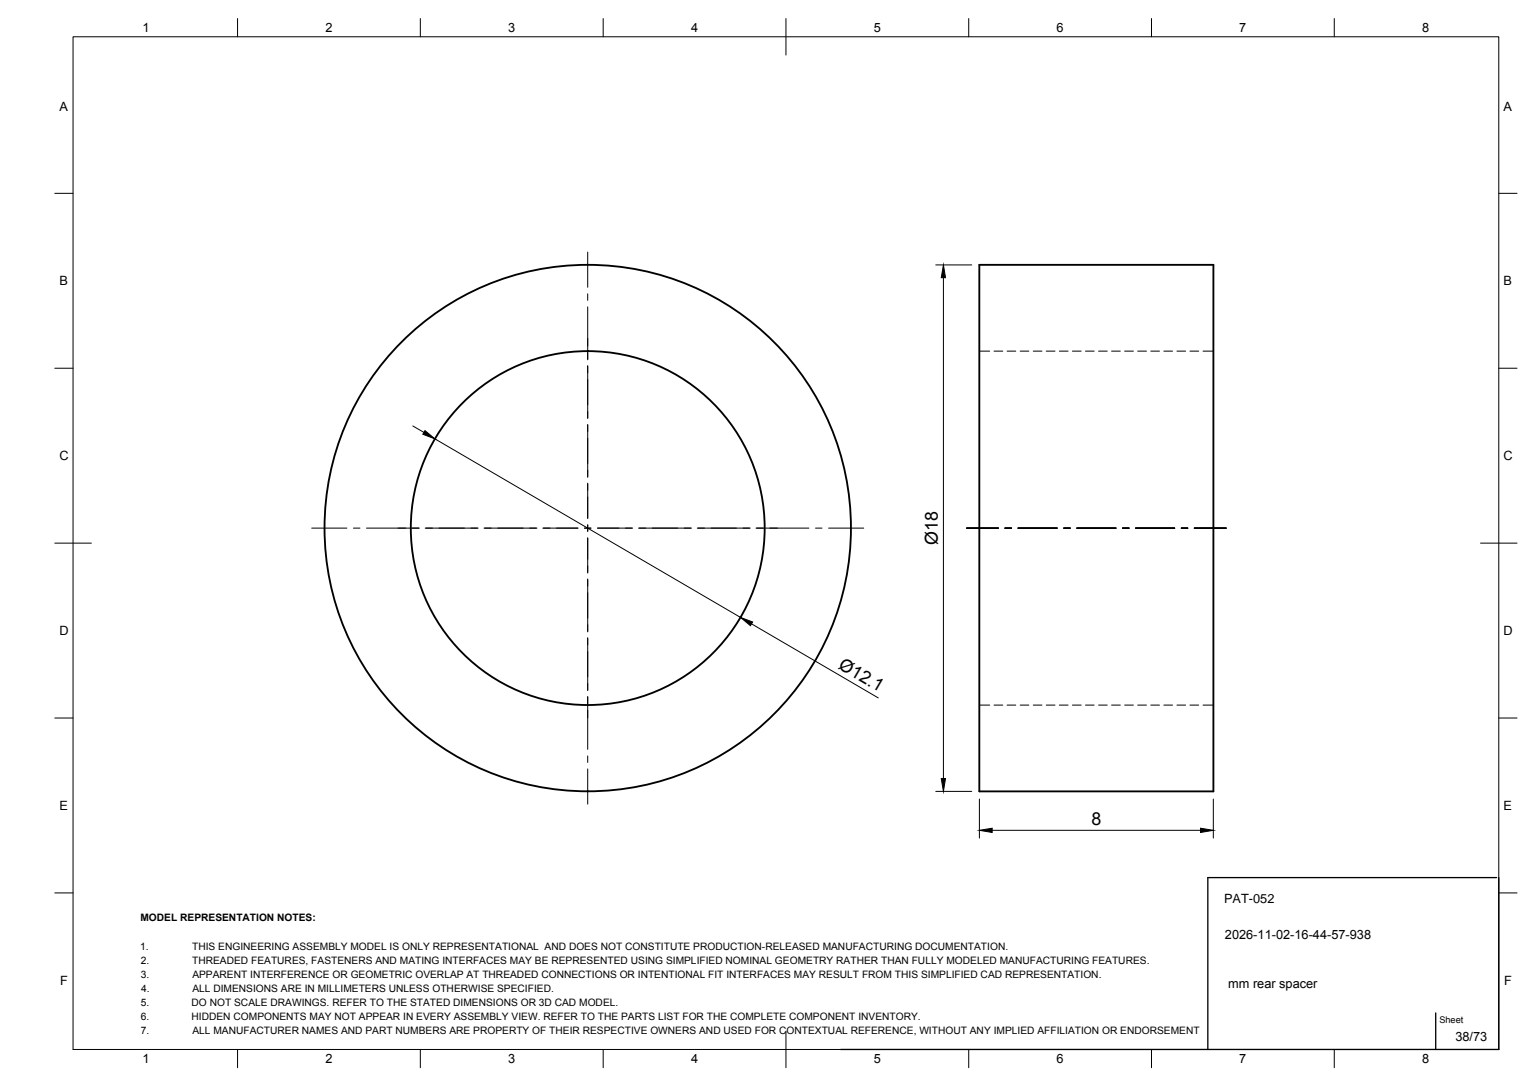
ISO-10303-21;
HEADER;
/* Generated by software containing ST-Developer
 * from STEP Tools, Inc. (www.steptools.com) 
 */

FILE_DESCRIPTION(
/* description */ ('Hand-crank gear train demonstrator'),
/* implementation_level */ '2;1');

FILE_NAME(
/* name */ 'mm rear spacer.step',
/* time_stamp */ '2026-10-28T03:22:13-07:00',
/* author */ (''),
/* organization */ (''),
/* preprocessor_version */ 'ST-DEVELOPER v20.2',
/* originating_system */ 'Autodesk Translation Framework v15.17.0.0',
/* authorisation */ '');

FILE_SCHEMA (('AUTOMOTIVE_DESIGN { 1 0 10303 214 3 1 1 }'));
ENDSEC;

DATA;
#10=MECHANICAL_DESIGN_GEOMETRIC_PRESENTATION_REPRESENTATION('',(#1234),#62758);
#1091=SHAPE_REPRESENTATION_RELATIONSHIP('SRR','None',#63066,#1155);
#1155=ADVANCED_BREP_SHAPE_REPRESENTATION('',(#1310),#62720);
#1234=STYLED_ITEM('',(#63476),#1310);
#1310=MANIFOLD_SOLID_BREP('Body1',#16417);
#1549=FACE_BOUND('',#3716,.T.);
#1550=FACE_BOUND('',#3718,.T.);
#1900=PLANE('',#18021);
#1901=PLANE('',#18022);
#2570=FACE_OUTER_BOUND('',#3713,.T.);
#2571=FACE_OUTER_BOUND('',#3714,.T.);
#2572=FACE_OUTER_BOUND('',#3715,.T.);
#2573=FACE_OUTER_BOUND('',#3717,.T.);
#3713=EDGE_LOOP('',(#12793,#12794,#12795,#12796));
#3714=EDGE_LOOP('',(#12797,#12798,#12799,#12800));
#3715=EDGE_LOOP('',(#12801));
#3716=EDGE_LOOP('',(#12802));
#3717=EDGE_LOOP('',(#12803));
#3718=EDGE_LOOP('',(#12804));
#4869=LINE('',#26084,#6001);
#4870=LINE('',#26090,#6002);
#6001=VECTOR('',#21132,0.605);
#6002=VECTOR('',#21139,0.9);
#6914=CIRCLE('',#18016,0.605);
#6915=CIRCLE('',#18017,0.605);
#6916=CIRCLE('',#18019,0.9);
#6917=CIRCLE('',#18020,0.9);
#7879=VERTEX_POINT('',#26081);
#7880=VERTEX_POINT('',#26083);
#7881=VERTEX_POINT('',#26087);
#7882=VERTEX_POINT('',#26089);
#9648=EDGE_CURVE('',#7879,#7879,#6914,.T.);
#9649=EDGE_CURVE('',#7879,#7880,#4869,.T.);
#9650=EDGE_CURVE('',#7880,#7880,#6915,.T.);
#9651=EDGE_CURVE('',#7881,#7881,#6916,.T.);
#9652=EDGE_CURVE('',#7881,#7882,#4870,.T.);
#9653=EDGE_CURVE('',#7882,#7882,#6917,.T.);
#12793=ORIENTED_EDGE('',*,*,#9648,.F.);
#12794=ORIENTED_EDGE('',*,*,#9649,.T.);
#12795=ORIENTED_EDGE('',*,*,#9650,.T.);
#12796=ORIENTED_EDGE('',*,*,#9649,.F.);
#12797=ORIENTED_EDGE('',*,*,#9651,.F.);
#12798=ORIENTED_EDGE('',*,*,#9652,.T.);
#12799=ORIENTED_EDGE('',*,*,#9653,.T.);
#12800=ORIENTED_EDGE('',*,*,#9652,.F.);
#12801=ORIENTED_EDGE('',*,*,#9651,.T.);
#12802=ORIENTED_EDGE('',*,*,#9648,.T.);
#12803=ORIENTED_EDGE('',*,*,#9653,.F.);
#12804=ORIENTED_EDGE('',*,*,#9650,.F.);
#15296=CYLINDRICAL_SURFACE('',#18015,0.605);
#15297=CYLINDRICAL_SURFACE('',#18018,0.9);
#15880=ADVANCED_FACE('',(#2570),#15296,.F.);
#15881=ADVANCED_FACE('',(#2571),#15297,.T.);
#15882=ADVANCED_FACE('',(#2572,#1549),#1900,.T.);
#15883=ADVANCED_FACE('',(#2573,#1550),#1901,.F.);
#16417=CLOSED_SHELL('',(#15880,#15881,#15882,#15883));
#18014=AXIS2_PLACEMENT_3D('',#26079,#21126,#21127);
#18015=AXIS2_PLACEMENT_3D('',#26080,#21128,#21129);
#18016=AXIS2_PLACEMENT_3D('',#26082,#21130,#21131);
#18017=AXIS2_PLACEMENT_3D('',#26085,#21133,#21134);
#18018=AXIS2_PLACEMENT_3D('',#26086,#21135,#21136);
#18019=AXIS2_PLACEMENT_3D('',#26088,#21137,#21138);
#18020=AXIS2_PLACEMENT_3D('',#26091,#21140,#21141);
#18021=AXIS2_PLACEMENT_3D('',#26092,#21142,#21143);
#18022=AXIS2_PLACEMENT_3D('',#26093,#21144,#21145);
#21126=DIRECTION('axis',(0.,0.,1.));
#21127=DIRECTION('refdir',(1.,0.,0.));
#21128=DIRECTION('center_axis',(0.,1.,0.));
#21129=DIRECTION('ref_axis',(1.,0.,0.));
#21130=DIRECTION('center_axis',(0.,-1.,0.));
#21131=DIRECTION('ref_axis',(1.,0.,0.));
#21132=DIRECTION('',(0.,-1.,0.));
#21133=DIRECTION('center_axis',(0.,-1.,0.));
#21134=DIRECTION('ref_axis',(1.,0.,0.));
#21135=DIRECTION('center_axis',(0.,1.,0.));
#21136=DIRECTION('ref_axis',(1.,0.,0.));
#21137=DIRECTION('center_axis',(0.,1.,0.));
#21138=DIRECTION('ref_axis',(1.,0.,0.));
#21139=DIRECTION('',(0.,-1.,0.));
#21140=DIRECTION('center_axis',(0.,1.,0.));
#21141=DIRECTION('ref_axis',(1.,0.,0.));
#21142=DIRECTION('center_axis',(0.,1.,0.));
#21143=DIRECTION('ref_axis',(1.,0.,0.));
#21144=DIRECTION('center_axis',(0.,1.,0.));
#21145=DIRECTION('ref_axis',(1.,0.,0.));
#26079=CARTESIAN_POINT('',(0.,0.,0.));
#26080=CARTESIAN_POINT('Origin',(0.,-2.8,9.));
#26081=CARTESIAN_POINT('',(-0.605,-2.,9.));
#26082=CARTESIAN_POINT('Origin',(0.,-2.,9.));
#26083=CARTESIAN_POINT('',(-0.605,-2.8,9.));
#26084=CARTESIAN_POINT('',(-0.605,-2.8,9.));
#26085=CARTESIAN_POINT('Origin',(0.,-2.8,9.));
#26086=CARTESIAN_POINT('Origin',(0.,-2.8,9.));
#26087=CARTESIAN_POINT('',(-0.9,-2.,9.));
#26088=CARTESIAN_POINT('Origin',(0.,-2.,9.));
#26089=CARTESIAN_POINT('',(-0.9,-2.8,9.));
#26090=CARTESIAN_POINT('',(-0.9,-2.8,9.));
#26091=CARTESIAN_POINT('Origin',(0.,-2.8,9.));
#26092=CARTESIAN_POINT('Origin',(0.,-2.,9.));
#26093=CARTESIAN_POINT('Origin',(0.,-2.8,9.));
#62646=UNCERTAINTY_MEASURE_WITH_UNIT(LENGTH_MEASURE(0.001),#62759,
'DISTANCE_ACCURACY_VALUE',
'Maximum model space distance between geometric entities at asserted c
onnectivities');
#62684=UNCERTAINTY_MEASURE_WITH_UNIT(LENGTH_MEASURE(0.001),#62759,
'DISTANCE_ACCURACY_VALUE',
'Maximum model space distance between geometric entities at asserted c
onnectivities');
#62720=(
GEOMETRIC_REPRESENTATION_CONTEXT(3)
GLOBAL_UNCERTAINTY_ASSIGNED_CONTEXT((#62646))
GLOBAL_UNIT_ASSIGNED_CONTEXT((#62759,#62761,#62762))
REPRESENTATION_CONTEXT('','3D')
);
#62758=(
GEOMETRIC_REPRESENTATION_CONTEXT(3)
GLOBAL_UNCERTAINTY_ASSIGNED_CONTEXT((#62684))
GLOBAL_UNIT_ASSIGNED_CONTEXT((#62759,#62761,#62762))
REPRESENTATION_CONTEXT('','3D')
);
#62759=(
LENGTH_UNIT()
NAMED_UNIT(*)
SI_UNIT(.CENTI.,.METRE.)
);
#62761=(
NAMED_UNIT(*)
PLANE_ANGLE_UNIT()
SI_UNIT($,.RADIAN.)
);
#62762=(
NAMED_UNIT(*)
SI_UNIT($,.STERADIAN.)
SOLID_ANGLE_UNIT()
);
#62798=SHAPE_DEFINITION_REPRESENTATION(#62881,#63066);
#62881=PRODUCT_DEFINITION_SHAPE('',$,#63140);
#63066=SHAPE_REPRESENTATION('',(#18014),#62720);
#63104=PRODUCT_DEFINITION_CONTEXT('part definition',#63325,'design');
#63140=PRODUCT_DEFINITION('mm rear spacer','mm rear spacer',#63213,#63104);
#63213=PRODUCT_DEFINITION_FORMATION('',$,#63362);
#63325=APPLICATION_CONTEXT(
'Core Data for Automotive Mechanical Design Process');
#63326=PRODUCT_CONTEXT('part definition',#63325,'mechanical');
#63362=PRODUCT('mm rear spacer','mm rear spacer','mm rear spacer',(#63326));
#63470=COLOUR_RGB('Off White',0.89,0.88,0.83);
#63471=FILL_AREA_STYLE_COLOUR('',#63470);
#63472=FILL_AREA_STYLE('',(#63471));
#63473=SURFACE_STYLE_FILL_AREA(#63472);
#63474=SURFACE_SIDE_STYLE('',(#63473));
#63475=SURFACE_STYLE_USAGE(.BOTH.,#63474);
#63476=PRESENTATION_STYLE_ASSIGNMENT((#63475));
ENDSEC;
END-ISO-10303-21;
